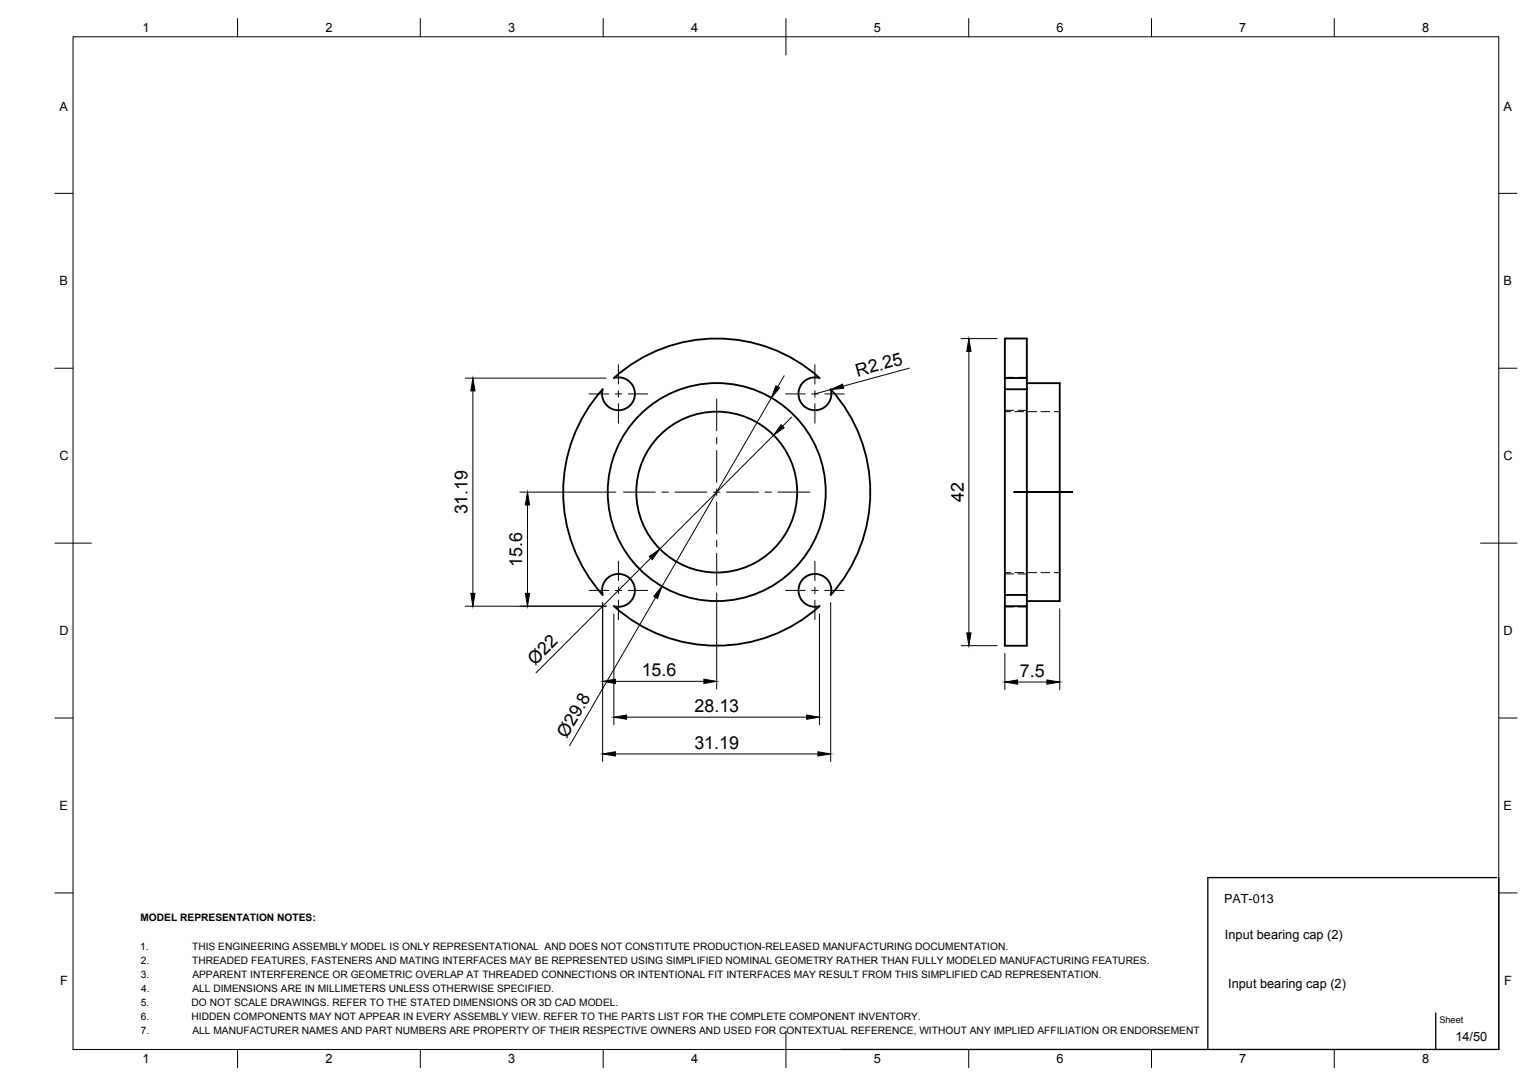
ISO-10303-21;
HEADER;
/* Generated by software containing ST-Developer
 * from STEP Tools, Inc. (www.steptools.com) 
 */

FILE_DESCRIPTION(
/* description */ ('Belt-driven linear axis on 2020 extrusion'),
/* implementation_level */ '2;1');

FILE_NAME(
/* name */ 'Input bearing cap (2).step',
/* time_stamp */ '2026-10-28T03:26:09-07:00',
/* author */ (''),
/* organization */ (''),
/* preprocessor_version */ 'ST-DEVELOPER v20.2',
/* originating_system */ 'Autodesk Translation Framework v15.17.0.0',
/* authorisation */ '');

FILE_SCHEMA (('AUTOMOTIVE_DESIGN { 1 0 10303 214 3 1 1 }'));
ENDSEC;

DATA;
#10=MECHANICAL_DESIGN_GEOMETRIC_PRESENTATION_REPRESENTATION('',(#621),#20096);
#527=SHAPE_REPRESENTATION_RELATIONSHIP('SRR','None',#20323,#573);
#573=ADVANCED_BREP_SHAPE_REPRESENTATION('',(#677),#20054);
#621=STYLED_ITEM('',(#20650),#677);
#677=MANIFOLD_SOLID_BREP('Body1',#10934);
#788=FACE_BOUND('',#2085,.T.);
#789=FACE_BOUND('',#2092,.T.);
#790=FACE_BOUND('',#2095,.T.);
#965=PLANE('',#11776);
#966=PLANE('',#11793);
#967=PLANE('',#11796);
#1388=FACE_OUTER_BOUND('',#2080,.T.);
#1389=FACE_OUTER_BOUND('',#2081,.T.);
#1390=FACE_OUTER_BOUND('',#2082,.T.);
#1391=FACE_OUTER_BOUND('',#2083,.T.);
#1392=FACE_OUTER_BOUND('',#2084,.T.);
#1393=FACE_OUTER_BOUND('',#2086,.T.);
#1394=FACE_OUTER_BOUND('',#2087,.T.);
#1395=FACE_OUTER_BOUND('',#2088,.T.);
#1396=FACE_OUTER_BOUND('',#2089,.T.);
#1397=FACE_OUTER_BOUND('',#2090,.T.);
#1398=FACE_OUTER_BOUND('',#2091,.T.);
#1399=FACE_OUTER_BOUND('',#2093,.T.);
#1400=FACE_OUTER_BOUND('',#2094,.T.);
#2080=EDGE_LOOP('',(#7841,#7842,#7843,#7844));
#2081=EDGE_LOOP('',(#7845,#7846,#7847,#7848));
#2082=EDGE_LOOP('',(#7849,#7850,#7851,#7852));
#2083=EDGE_LOOP('',(#7853,#7854,#7855,#7856));
#2084=EDGE_LOOP('',(#7857,#7858,#7859,#7860,#7861,#7862,#7863,#7864));
#2085=EDGE_LOOP('',(#7865));
#2086=EDGE_LOOP('',(#7866,#7867,#7868,#7869));
#2087=EDGE_LOOP('',(#7870,#7871,#7872,#7873));
#2088=EDGE_LOOP('',(#7874,#7875,#7876,#7877));
#2089=EDGE_LOOP('',(#7878,#7879,#7880,#7881));
#2090=EDGE_LOOP('',(#7882,#7883,#7884,#7885));
#2091=EDGE_LOOP('',(#7886));
#2092=EDGE_LOOP('',(#7887));
#2093=EDGE_LOOP('',(#7888,#7889,#7890,#7891));
#2094=EDGE_LOOP('',(#7892,#7893,#7894,#7895,#7896,#7897,#7898,#7899));
#2095=EDGE_LOOP('',(#7900));
#2835=LINE('',#16875,#3692);
#2836=LINE('',#16879,#3693);
#2837=LINE('',#16884,#3694);
#2838=LINE('',#16888,#3695);
#2839=LINE('',#16893,#3696);
#2840=LINE('',#16897,#3697);
#2841=LINE('',#16902,#3698);
#2842=LINE('',#16906,#3699);
#2843=LINE('',#16927,#3700);
#2844=LINE('',#16933,#3701);
#3692=VECTOR('',#13505,1.);
#3693=VECTOR('',#13508,1.);
#3694=VECTOR('',#13513,1.);
#3695=VECTOR('',#13516,1.);
#3696=VECTOR('',#13521,1.);
#3697=VECTOR('',#13524,1.);
#3698=VECTOR('',#13529,1.);
#3699=VECTOR('',#13532,1.);
#3700=VECTOR('',#13567,1.49);
#3701=VECTOR('',#13576,1.1);
#4503=CIRCLE('',#11765,0.225000000000001);
#4504=CIRCLE('',#11766,0.225000000000001);
#4505=CIRCLE('',#11768,0.225000000000001);
#4506=CIRCLE('',#11769,0.225000000000001);
#4507=CIRCLE('',#11771,0.225000000000001);
#4508=CIRCLE('',#11772,0.225000000000001);
#4509=CIRCLE('',#11774,0.225000000000001);
#4510=CIRCLE('',#11775,0.225000000000001);
#4511=CIRCLE('',#11777,2.1);
#4512=CIRCLE('',#11778,2.1);
#4513=CIRCLE('',#11779,2.1);
#4514=CIRCLE('',#11780,2.1);
#4515=CIRCLE('',#11781,1.1);
#4516=CIRCLE('',#11783,2.1);
#4517=CIRCLE('',#11785,2.1);
#4518=CIRCLE('',#11787,2.1);
#4519=CIRCLE('',#11789,2.1);
#4520=CIRCLE('',#11791,1.49);
#4521=CIRCLE('',#11792,1.49);
#4522=CIRCLE('',#11794,1.1);
#5088=VERTEX_POINT('',#16873);
#5089=VERTEX_POINT('',#16874);
#5090=VERTEX_POINT('',#16876);
#5091=VERTEX_POINT('',#16878);
#5092=VERTEX_POINT('',#16882);
#5093=VERTEX_POINT('',#16883);
#5094=VERTEX_POINT('',#16885);
#5095=VERTEX_POINT('',#16887);
#5096=VERTEX_POINT('',#16891);
#5097=VERTEX_POINT('',#16892);
#5098=VERTEX_POINT('',#16894);
#5099=VERTEX_POINT('',#16896);
#5100=VERTEX_POINT('',#16900);
#5101=VERTEX_POINT('',#16901);
#5102=VERTEX_POINT('',#16903);
#5103=VERTEX_POINT('',#16905);
#5104=VERTEX_POINT('',#16913);
#5105=VERTEX_POINT('',#16924);
#5106=VERTEX_POINT('',#16926);
#5107=VERTEX_POINT('',#16930);
#6135=EDGE_CURVE('',#5088,#5089,#2835,.T.);
#6136=EDGE_CURVE('',#5090,#5088,#4503,.T.);
#6137=EDGE_CURVE('',#5091,#5090,#2836,.T.);
#6138=EDGE_CURVE('',#5089,#5091,#4504,.T.);
#6139=EDGE_CURVE('',#5092,#5093,#2837,.T.);
#6140=EDGE_CURVE('',#5094,#5092,#4505,.T.);
#6141=EDGE_CURVE('',#5095,#5094,#2838,.T.);
#6142=EDGE_CURVE('',#5093,#5095,#4506,.T.);
#6143=EDGE_CURVE('',#5096,#5097,#2839,.T.);
#6144=EDGE_CURVE('',#5098,#5096,#4507,.T.);
#6145=EDGE_CURVE('',#5099,#5098,#2840,.T.);
#6146=EDGE_CURVE('',#5097,#5099,#4508,.T.);
#6147=EDGE_CURVE('',#5100,#5101,#2841,.T.);
#6148=EDGE_CURVE('',#5102,#5100,#4509,.T.);
#6149=EDGE_CURVE('',#5103,#5102,#2842,.T.);
#6150=EDGE_CURVE('',#5101,#5103,#4510,.T.);
#6151=EDGE_CURVE('',#5102,#5088,#4511,.T.);
#6152=EDGE_CURVE('',#5098,#5100,#4512,.T.);
#6153=EDGE_CURVE('',#5094,#5096,#4513,.T.);
#6154=EDGE_CURVE('',#5090,#5092,#4514,.T.);
#6155=EDGE_CURVE('',#5104,#5104,#4515,.T.);
#6156=EDGE_CURVE('',#5099,#5101,#4516,.T.);
#6157=EDGE_CURVE('',#5095,#5097,#4517,.T.);
#6158=EDGE_CURVE('',#5103,#5089,#4518,.T.);
#6159=EDGE_CURVE('',#5091,#5093,#4519,.T.);
#6160=EDGE_CURVE('',#5105,#5105,#4520,.T.);
#6161=EDGE_CURVE('',#5105,#5106,#2843,.T.);
#6162=EDGE_CURVE('',#5106,#5106,#4521,.T.);
#6163=EDGE_CURVE('',#5107,#5107,#4522,.T.);
#6164=EDGE_CURVE('',#5107,#5104,#2844,.T.);
#7841=ORIENTED_EDGE('',*,*,#6135,.F.);
#7842=ORIENTED_EDGE('',*,*,#6136,.F.);
#7843=ORIENTED_EDGE('',*,*,#6137,.F.);
#7844=ORIENTED_EDGE('',*,*,#6138,.F.);
#7845=ORIENTED_EDGE('',*,*,#6139,.F.);
#7846=ORIENTED_EDGE('',*,*,#6140,.F.);
#7847=ORIENTED_EDGE('',*,*,#6141,.F.);
#7848=ORIENTED_EDGE('',*,*,#6142,.F.);
#7849=ORIENTED_EDGE('',*,*,#6143,.F.);
#7850=ORIENTED_EDGE('',*,*,#6144,.F.);
#7851=ORIENTED_EDGE('',*,*,#6145,.F.);
#7852=ORIENTED_EDGE('',*,*,#6146,.F.);
#7853=ORIENTED_EDGE('',*,*,#6147,.F.);
#7854=ORIENTED_EDGE('',*,*,#6148,.F.);
#7855=ORIENTED_EDGE('',*,*,#6149,.F.);
#7856=ORIENTED_EDGE('',*,*,#6150,.F.);
#7857=ORIENTED_EDGE('',*,*,#6136,.T.);
#7858=ORIENTED_EDGE('',*,*,#6151,.F.);
#7859=ORIENTED_EDGE('',*,*,#6148,.T.);
#7860=ORIENTED_EDGE('',*,*,#6152,.F.);
#7861=ORIENTED_EDGE('',*,*,#6144,.T.);
#7862=ORIENTED_EDGE('',*,*,#6153,.F.);
#7863=ORIENTED_EDGE('',*,*,#6140,.T.);
#7864=ORIENTED_EDGE('',*,*,#6154,.F.);
#7865=ORIENTED_EDGE('',*,*,#6155,.F.);
#7866=ORIENTED_EDGE('',*,*,#6145,.T.);
#7867=ORIENTED_EDGE('',*,*,#6152,.T.);
#7868=ORIENTED_EDGE('',*,*,#6147,.T.);
#7869=ORIENTED_EDGE('',*,*,#6156,.F.);
#7870=ORIENTED_EDGE('',*,*,#6141,.T.);
#7871=ORIENTED_EDGE('',*,*,#6153,.T.);
#7872=ORIENTED_EDGE('',*,*,#6143,.T.);
#7873=ORIENTED_EDGE('',*,*,#6157,.F.);
#7874=ORIENTED_EDGE('',*,*,#6135,.T.);
#7875=ORIENTED_EDGE('',*,*,#6158,.F.);
#7876=ORIENTED_EDGE('',*,*,#6149,.T.);
#7877=ORIENTED_EDGE('',*,*,#6151,.T.);
#7878=ORIENTED_EDGE('',*,*,#6137,.T.);
#7879=ORIENTED_EDGE('',*,*,#6154,.T.);
#7880=ORIENTED_EDGE('',*,*,#6139,.T.);
#7881=ORIENTED_EDGE('',*,*,#6159,.F.);
#7882=ORIENTED_EDGE('',*,*,#6160,.F.);
#7883=ORIENTED_EDGE('',*,*,#6161,.T.);
#7884=ORIENTED_EDGE('',*,*,#6162,.F.);
#7885=ORIENTED_EDGE('',*,*,#6161,.F.);
#7886=ORIENTED_EDGE('',*,*,#6160,.T.);
#7887=ORIENTED_EDGE('',*,*,#6163,.T.);
#7888=ORIENTED_EDGE('',*,*,#6163,.F.);
#7889=ORIENTED_EDGE('',*,*,#6164,.T.);
#7890=ORIENTED_EDGE('',*,*,#6155,.T.);
#7891=ORIENTED_EDGE('',*,*,#6164,.F.);
#7892=ORIENTED_EDGE('',*,*,#6138,.T.);
#7893=ORIENTED_EDGE('',*,*,#6159,.T.);
#7894=ORIENTED_EDGE('',*,*,#6142,.T.);
#7895=ORIENTED_EDGE('',*,*,#6157,.T.);
#7896=ORIENTED_EDGE('',*,*,#6146,.T.);
#7897=ORIENTED_EDGE('',*,*,#6156,.T.);
#7898=ORIENTED_EDGE('',*,*,#6150,.T.);
#7899=ORIENTED_EDGE('',*,*,#6158,.T.);
#7900=ORIENTED_EDGE('',*,*,#6162,.T.);
#10139=CYLINDRICAL_SURFACE('',#11764,0.225000000000001);
#10140=CYLINDRICAL_SURFACE('',#11767,0.225000000000001);
#10141=CYLINDRICAL_SURFACE('',#11770,0.225000000000001);
#10142=CYLINDRICAL_SURFACE('',#11773,0.225000000000001);
#10143=CYLINDRICAL_SURFACE('',#11782,2.1);
#10144=CYLINDRICAL_SURFACE('',#11784,2.1);
#10145=CYLINDRICAL_SURFACE('',#11786,2.1);
#10146=CYLINDRICAL_SURFACE('',#11788,2.1);
#10147=CYLINDRICAL_SURFACE('',#11790,1.49);
#10148=CYLINDRICAL_SURFACE('',#11795,1.1);
#10439=ADVANCED_FACE('',(#1388),#10139,.F.);
#10440=ADVANCED_FACE('',(#1389),#10140,.F.);
#10441=ADVANCED_FACE('',(#1390),#10141,.F.);
#10442=ADVANCED_FACE('',(#1391),#10142,.F.);
#10443=ADVANCED_FACE('',(#1392,#788),#965,.F.);
#10444=ADVANCED_FACE('',(#1393),#10143,.T.);
#10445=ADVANCED_FACE('',(#1394),#10144,.T.);
#10446=ADVANCED_FACE('',(#1395),#10145,.T.);
#10447=ADVANCED_FACE('',(#1396),#10146,.T.);
#10448=ADVANCED_FACE('',(#1397),#10147,.T.);
#10449=ADVANCED_FACE('',(#1398,#789),#966,.T.);
#10450=ADVANCED_FACE('',(#1399),#10148,.F.);
#10451=ADVANCED_FACE('',(#1400,#790),#967,.T.);
#10934=CLOSED_SHELL('',(#10439,#10440,#10441,#10442,#10443,#10444,#10445,
#10446,#10447,#10448,#10449,#10450,#10451));
#11763=AXIS2_PLACEMENT_3D('',#16871,#13501,#13502);
#11764=AXIS2_PLACEMENT_3D('',#16872,#13503,#13504);
#11765=AXIS2_PLACEMENT_3D('',#16877,#13506,#13507);
#11766=AXIS2_PLACEMENT_3D('',#16880,#13509,#13510);
#11767=AXIS2_PLACEMENT_3D('',#16881,#13511,#13512);
#11768=AXIS2_PLACEMENT_3D('',#16886,#13514,#13515);
#11769=AXIS2_PLACEMENT_3D('',#16889,#13517,#13518);
#11770=AXIS2_PLACEMENT_3D('',#16890,#13519,#13520);
#11771=AXIS2_PLACEMENT_3D('',#16895,#13522,#13523);
#11772=AXIS2_PLACEMENT_3D('',#16898,#13525,#13526);
#11773=AXIS2_PLACEMENT_3D('',#16899,#13527,#13528);
#11774=AXIS2_PLACEMENT_3D('',#16904,#13530,#13531);
#11775=AXIS2_PLACEMENT_3D('',#16907,#13533,#13534);
#11776=AXIS2_PLACEMENT_3D('',#16908,#13535,#13536);
#11777=AXIS2_PLACEMENT_3D('',#16909,#13537,#13538);
#11778=AXIS2_PLACEMENT_3D('',#16910,#13539,#13540);
#11779=AXIS2_PLACEMENT_3D('',#16911,#13541,#13542);
#11780=AXIS2_PLACEMENT_3D('',#16912,#13543,#13544);
#11781=AXIS2_PLACEMENT_3D('',#16914,#13545,#13546);
#11782=AXIS2_PLACEMENT_3D('',#16915,#13547,#13548);
#11783=AXIS2_PLACEMENT_3D('',#16916,#13549,#13550);
#11784=AXIS2_PLACEMENT_3D('',#16917,#13551,#13552);
#11785=AXIS2_PLACEMENT_3D('',#16918,#13553,#13554);
#11786=AXIS2_PLACEMENT_3D('',#16919,#13555,#13556);
#11787=AXIS2_PLACEMENT_3D('',#16920,#13557,#13558);
#11788=AXIS2_PLACEMENT_3D('',#16921,#13559,#13560);
#11789=AXIS2_PLACEMENT_3D('',#16922,#13561,#13562);
#11790=AXIS2_PLACEMENT_3D('',#16923,#13563,#13564);
#11791=AXIS2_PLACEMENT_3D('',#16925,#13565,#13566);
#11792=AXIS2_PLACEMENT_3D('',#16928,#13568,#13569);
#11793=AXIS2_PLACEMENT_3D('',#16929,#13570,#13571);
#11794=AXIS2_PLACEMENT_3D('',#16931,#13572,#13573);
#11795=AXIS2_PLACEMENT_3D('',#16932,#13574,#13575);
#11796=AXIS2_PLACEMENT_3D('',#16934,#13577,#13578);
#13501=DIRECTION('axis',(0.,0.,1.));
#13502=DIRECTION('refdir',(1.,0.,0.));
#13503=DIRECTION('center_axis',(0.,1.,0.));
#13504=DIRECTION('ref_axis',(0.70710678118656,0.,0.707106781186535));
#13505=DIRECTION('',(0.,1.,0.));
#13506=DIRECTION('center_axis',(0.,1.,0.));
#13507=DIRECTION('ref_axis',(1.,0.,0.));
#13508=DIRECTION('',(0.,-1.,0.));
#13509=DIRECTION('center_axis',(0.,-1.,0.));
#13510=DIRECTION('ref_axis',(1.,0.,0.));
#13511=DIRECTION('center_axis',(0.,1.,0.));
#13512=DIRECTION('ref_axis',(0.707106781186561,0.,-0.707106781186534));
#13513=DIRECTION('',(0.,1.,0.));
#13514=DIRECTION('center_axis',(0.,1.,0.));
#13515=DIRECTION('ref_axis',(1.,0.,0.));
#13516=DIRECTION('',(0.,-1.,0.));
#13517=DIRECTION('center_axis',(0.,-1.,0.));
#13518=DIRECTION('ref_axis',(1.,0.,0.));
#13519=DIRECTION('center_axis',(0.,1.,0.));
#13520=DIRECTION('ref_axis',(-0.707106781186554,0.,-0.707106781186541));
#13521=DIRECTION('',(0.,1.,0.));
#13522=DIRECTION('center_axis',(0.,1.,0.));
#13523=DIRECTION('ref_axis',(1.,0.,0.));
#13524=DIRECTION('',(0.,-1.,0.));
#13525=DIRECTION('center_axis',(0.,-1.,0.));
#13526=DIRECTION('ref_axis',(1.,0.,0.));
#13527=DIRECTION('center_axis',(0.,1.,0.));
#13528=DIRECTION('ref_axis',(-0.707106781186554,0.,0.707106781186541));
#13529=DIRECTION('',(0.,1.,0.));
#13530=DIRECTION('center_axis',(0.,1.,0.));
#13531=DIRECTION('ref_axis',(1.,0.,0.));
#13532=DIRECTION('',(0.,-1.,0.));
#13533=DIRECTION('center_axis',(0.,-1.,0.));
#13534=DIRECTION('ref_axis',(1.,0.,0.));
#13535=DIRECTION('center_axis',(0.,1.,0.));
#13536=DIRECTION('ref_axis',(1.,0.,0.));
#13537=DIRECTION('center_axis',(0.,1.,0.));
#13538=DIRECTION('ref_axis',(1.,0.,0.));
#13539=DIRECTION('center_axis',(0.,1.,0.));
#13540=DIRECTION('ref_axis',(1.,0.,0.));
#13541=DIRECTION('center_axis',(0.,1.,0.));
#13542=DIRECTION('ref_axis',(1.,0.,0.));
#13543=DIRECTION('center_axis',(0.,1.,0.));
#13544=DIRECTION('ref_axis',(1.,0.,0.));
#13545=DIRECTION('center_axis',(0.,-1.,0.));
#13546=DIRECTION('ref_axis',(1.,0.,0.));
#13547=DIRECTION('center_axis',(0.,1.,0.));
#13548=DIRECTION('ref_axis',(1.,0.,0.));
#13549=DIRECTION('center_axis',(0.,1.,0.));
#13550=DIRECTION('ref_axis',(1.,0.,0.));
#13551=DIRECTION('center_axis',(0.,1.,0.));
#13552=DIRECTION('ref_axis',(1.,0.,0.));
#13553=DIRECTION('center_axis',(0.,1.,0.));
#13554=DIRECTION('ref_axis',(1.,0.,0.));
#13555=DIRECTION('center_axis',(0.,1.,0.));
#13556=DIRECTION('ref_axis',(1.,0.,0.));
#13557=DIRECTION('center_axis',(0.,1.,0.));
#13558=DIRECTION('ref_axis',(1.,0.,0.));
#13559=DIRECTION('center_axis',(0.,1.,0.));
#13560=DIRECTION('ref_axis',(-1.,0.,-1.22464679914735E-16));
#13561=DIRECTION('center_axis',(0.,1.,0.));
#13562=DIRECTION('ref_axis',(1.,0.,0.));
#13563=DIRECTION('center_axis',(0.,1.,0.));
#13564=DIRECTION('ref_axis',(1.,0.,0.));
#13565=DIRECTION('center_axis',(0.,1.,0.));
#13566=DIRECTION('ref_axis',(1.,0.,0.));
#13567=DIRECTION('',(0.,-1.,0.));
#13568=DIRECTION('center_axis',(0.,-1.,0.));
#13569=DIRECTION('ref_axis',(1.,0.,0.));
#13570=DIRECTION('center_axis',(0.,1.,0.));
#13571=DIRECTION('ref_axis',(1.,0.,0.));
#13572=DIRECTION('center_axis',(0.,-1.,0.));
#13573=DIRECTION('ref_axis',(1.,0.,0.));
#13574=DIRECTION('center_axis',(0.,1.,0.));
#13575=DIRECTION('ref_axis',(1.,0.,0.));
#13576=DIRECTION('',(0.,-1.,0.));
#13577=DIRECTION('center_axis',(0.,1.,0.));
#13578=DIRECTION('ref_axis',(1.,0.,0.));
#16871=CARTESIAN_POINT('',(0.,0.,0.));
#16872=CARTESIAN_POINT('Origin',(30.6564971157456,-2.2,5.65649711574556));
#16873=CARTESIAN_POINT('',(30.5936544441036,-2.1,5.4404512904656));
#16874=CARTESIAN_POINT('',(30.5936544441036,-1.8,5.4404512904656));
#16875=CARTESIAN_POINT('',(30.5936544441036,-2.2,5.4404512904656));
#16876=CARTESIAN_POINT('',(30.4404512904656,-2.1,5.59365444410359));
#16877=CARTESIAN_POINT('Origin',(30.6564971157456,-2.1,5.65649711574556));
#16878=CARTESIAN_POINT('',(30.4404512904656,-1.8,5.59365444410359));
#16879=CARTESIAN_POINT('',(30.4404512904656,-2.2,5.59365444410359));
#16880=CARTESIAN_POINT('Origin',(30.6564971157456,-1.8,5.65649711574556));
#16881=CARTESIAN_POINT('Origin',(30.6564971157456,-2.2,8.34350288425444));
#16882=CARTESIAN_POINT('',(30.4404512904656,-2.1,8.40634555589641));
#16883=CARTESIAN_POINT('',(30.4404512904656,-1.8,8.40634555589641));
#16884=CARTESIAN_POINT('',(30.4404512904656,-2.2,8.40634555589641));
#16885=CARTESIAN_POINT('',(30.5936544441036,-2.1,8.5595487095344));
#16886=CARTESIAN_POINT('Origin',(30.6564971157456,-2.1,8.34350288425444));
#16887=CARTESIAN_POINT('',(30.5936544441036,-1.8,8.5595487095344));
#16888=CARTESIAN_POINT('',(30.5936544441036,-2.2,8.5595487095344));
#16889=CARTESIAN_POINT('Origin',(30.6564971157456,-1.8,8.34350288425444));
#16890=CARTESIAN_POINT('Origin',(33.3435028842544,-2.2,8.34350288425444));
#16891=CARTESIAN_POINT('',(33.4063455558964,-2.1,8.5595487095344));
#16892=CARTESIAN_POINT('',(33.4063455558964,-1.8,8.5595487095344));
#16893=CARTESIAN_POINT('',(33.4063455558964,-2.2,8.5595487095344));
#16894=CARTESIAN_POINT('',(33.5595487095344,-2.1,8.40634555589641));
#16895=CARTESIAN_POINT('Origin',(33.3435028842544,-2.1,8.34350288425444));
#16896=CARTESIAN_POINT('',(33.5595487095344,-1.8,8.40634555589641));
#16897=CARTESIAN_POINT('',(33.5595487095344,-2.2,8.40634555589641));
#16898=CARTESIAN_POINT('Origin',(33.3435028842544,-1.8,8.34350288425444));
#16899=CARTESIAN_POINT('Origin',(33.3435028842544,-2.2,5.65649711574556));
#16900=CARTESIAN_POINT('',(33.5595487095344,-2.1,5.59365444410359));
#16901=CARTESIAN_POINT('',(33.5595487095344,-1.8,5.59365444410359));
#16902=CARTESIAN_POINT('',(33.5595487095344,-2.2,5.59365444410359));
#16903=CARTESIAN_POINT('',(33.4063455558964,-2.1,5.4404512904656));
#16904=CARTESIAN_POINT('Origin',(33.3435028842544,-2.1,5.65649711574556));
#16905=CARTESIAN_POINT('',(33.4063455558964,-1.8,5.4404512904656));
#16906=CARTESIAN_POINT('',(33.4063455558964,-2.2,5.4404512904656));
#16907=CARTESIAN_POINT('Origin',(33.3435028842544,-1.8,5.65649711574556));
#16908=CARTESIAN_POINT('Origin',(32.,-2.1,7.));
#16909=CARTESIAN_POINT('Origin',(32.,-2.1,7.));
#16910=CARTESIAN_POINT('Origin',(32.,-2.1,7.));
#16911=CARTESIAN_POINT('Origin',(32.,-2.1,7.));
#16912=CARTESIAN_POINT('Origin',(32.,-2.1,7.));
#16913=CARTESIAN_POINT('',(30.9,-2.1,7.));
#16914=CARTESIAN_POINT('Origin',(32.,-2.1,7.));
#16915=CARTESIAN_POINT('Origin',(32.,-2.1,7.));
#16916=CARTESIAN_POINT('Origin',(32.,-1.8,7.));
#16917=CARTESIAN_POINT('Origin',(32.,-2.1,7.));
#16918=CARTESIAN_POINT('Origin',(32.,-1.8,7.));
#16919=CARTESIAN_POINT('Origin',(32.,-2.1,7.));
#16920=CARTESIAN_POINT('Origin',(32.,-1.8,7.));
#16921=CARTESIAN_POINT('Origin',(32.,-2.1,7.));
#16922=CARTESIAN_POINT('Origin',(32.,-1.8,7.));
#16923=CARTESIAN_POINT('Origin',(32.,-1.8,7.));
#16924=CARTESIAN_POINT('',(30.51,-1.35,7.));
#16925=CARTESIAN_POINT('Origin',(32.,-1.35,7.));
#16926=CARTESIAN_POINT('',(30.51,-1.8,7.));
#16927=CARTESIAN_POINT('',(30.51,-1.8,7.));
#16928=CARTESIAN_POINT('Origin',(32.,-1.8,7.));
#16929=CARTESIAN_POINT('Origin',(32.,-1.35,7.));
#16930=CARTESIAN_POINT('',(30.9,-1.35,7.));
#16931=CARTESIAN_POINT('Origin',(32.,-1.35,7.));
#16932=CARTESIAN_POINT('Origin',(32.,-2.1,7.));
#16933=CARTESIAN_POINT('',(30.9,-2.1,7.));
#16934=CARTESIAN_POINT('Origin',(32.,-1.8,7.));
#20000=UNCERTAINTY_MEASURE_WITH_UNIT(LENGTH_MEASURE(0.001),#20097,
'DISTANCE_ACCURACY_VALUE',
'Maximum model space distance between geometric entities at asserted c
onnectivities');
#20042=UNCERTAINTY_MEASURE_WITH_UNIT(LENGTH_MEASURE(0.001),#20097,
'DISTANCE_ACCURACY_VALUE',
'Maximum model space distance between geometric entities at asserted c
onnectivities');
#20054=(
GEOMETRIC_REPRESENTATION_CONTEXT(3)
GLOBAL_UNCERTAINTY_ASSIGNED_CONTEXT((#20000))
GLOBAL_UNIT_ASSIGNED_CONTEXT((#20097,#20099,#20100))
REPRESENTATION_CONTEXT('','3D')
);
#20096=(
GEOMETRIC_REPRESENTATION_CONTEXT(3)
GLOBAL_UNCERTAINTY_ASSIGNED_CONTEXT((#20042))
GLOBAL_UNIT_ASSIGNED_CONTEXT((#20097,#20099,#20100))
REPRESENTATION_CONTEXT('','3D')
);
#20097=(
LENGTH_UNIT()
NAMED_UNIT(*)
SI_UNIT(.CENTI.,.METRE.)
);
#20099=(
NAMED_UNIT(*)
PLANE_ANGLE_UNIT()
SI_UNIT($,.RADIAN.)
);
#20100=(
NAMED_UNIT(*)
SI_UNIT($,.STERADIAN.)
SOLID_ANGLE_UNIT()
);
#20112=SHAPE_DEFINITION_REPRESENTATION(#20165,#20323);
#20165=PRODUCT_DEFINITION_SHAPE('',$,#20377);
#20323=SHAPE_REPRESENTATION('',(#11763),#20054);
#20365=PRODUCT_DEFINITION_CONTEXT('part definition',#20526,'design');
#20377=PRODUCT_DEFINITION('Input bearing cap (2)','Input bearing cap (2)',
#20430,#20365);
#20430=PRODUCT_DEFINITION_FORMATION('',$,#20539);
#20526=APPLICATION_CONTEXT(
'Core Data for Automotive Mechanical Design Process');
#20527=PRODUCT_CONTEXT('part definition',#20526,'mechanical');
#20539=PRODUCT('Input bearing cap (2)','Input bearing cap (2)',
'Input bearing cap (2)',(#20527));
#20644=COLOUR_RGB('Grey',0.48,0.52,0.57);
#20645=FILL_AREA_STYLE_COLOUR('',#20644);
#20646=FILL_AREA_STYLE('',(#20645));
#20647=SURFACE_STYLE_FILL_AREA(#20646);
#20648=SURFACE_SIDE_STYLE('',(#20647));
#20649=SURFACE_STYLE_USAGE(.BOTH.,#20648);
#20650=PRESENTATION_STYLE_ASSIGNMENT((#20649));
ENDSEC;
END-ISO-10303-21;
